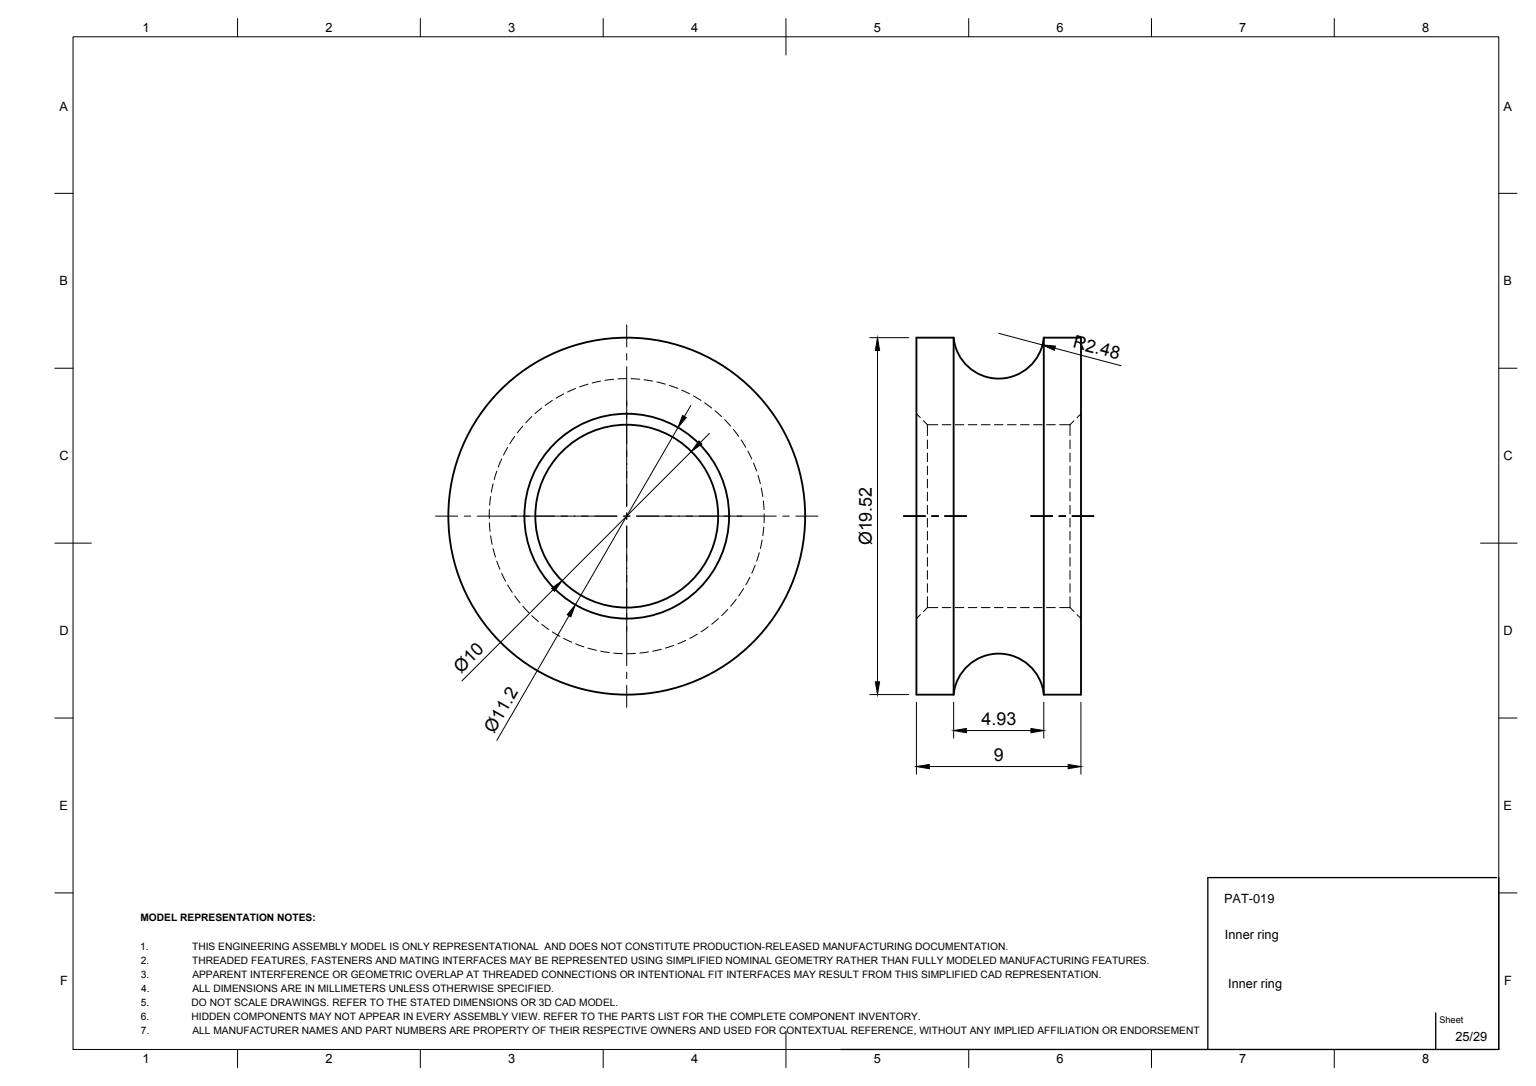
ISO-10303-21;
HEADER;
/* Generated by software containing ST-Developer
 * from STEP Tools, Inc. (www.steptools.com) 
 */

FILE_DESCRIPTION(
/* description */ ('Caster wheel assembly'),
/* implementation_level */ '2;1');

FILE_NAME(
/* name */ 'Inner ring.step',
/* time_stamp */ '2026-10-28T03:23:56-07:00',
/* author */ (''),
/* organization */ (''),
/* preprocessor_version */ 'ST-DEVELOPER v20.2',
/* originating_system */ 'Autodesk Translation Framework v15.17.0.0',
/* authorisation */ '');

FILE_SCHEMA (('AUTOMOTIVE_DESIGN { 1 0 10303 214 3 1 1 }'));
ENDSEC;

DATA;
#10=MECHANICAL_DESIGN_GEOMETRIC_PRESENTATION_REPRESENTATION('',(#239),#5385);
#45=TOROIDAL_SURFACE('',#3164,1.,0.247676);
#174=CONICAL_SURFACE('',#3175,0.53,0.785398163397448);
#175=CONICAL_SURFACE('',#3182,0.53,0.785398163397448);
#195=SHAPE_REPRESENTATION_RELATIONSHIP('SRR','None',#5493,#217);
#217=ADVANCED_BREP_SHAPE_REPRESENTATION('',(#268),#5380);
#239=STYLED_ITEM('',(#5672),#268);
#268=MANIFOLD_SOLID_BREP('Body1',#2667);
#324=FACE_BOUND('',#754,.T.);
#325=FACE_BOUND('',#757,.T.);
#404=PLANE('',#3177);
#405=PLANE('',#3180);
#538=FACE_OUTER_BOUND('',#749,.T.);
#539=FACE_OUTER_BOUND('',#750,.T.);
#540=FACE_OUTER_BOUND('',#751,.T.);
#541=FACE_OUTER_BOUND('',#752,.T.);
#542=FACE_OUTER_BOUND('',#753,.T.);
#543=FACE_OUTER_BOUND('',#755,.T.);
#544=FACE_OUTER_BOUND('',#756,.T.);
#545=FACE_OUTER_BOUND('',#758,.T.);
#749=EDGE_LOOP('',(#2216,#2217,#2218,#2219,#2220,#2221));
#750=EDGE_LOOP('',(#2222,#2223,#2224,#2225,#2226));
#751=EDGE_LOOP('',(#2227,#2228,#2229,#2230));
#752=EDGE_LOOP('',(#2231,#2232,#2233,#2234));
#753=EDGE_LOOP('',(#2235));
#754=EDGE_LOOP('',(#2236));
#755=EDGE_LOOP('',(#2237,#2238,#2239,#2240,#2241));
#756=EDGE_LOOP('',(#2242));
#757=EDGE_LOOP('',(#2243));
#758=EDGE_LOOP('',(#2244,#2245,#2246,#2247));
#927=LINE('',#4750,#1061);
#928=LINE('',#4756,#1062);
#929=LINE('',#4760,#1063);
#930=LINE('',#4766,#1064);
#931=LINE('',#4771,#1065);
#1061=VECTOR('',#3918,0.976185);
#1062=VECTOR('',#3925,0.5);
#1063=VECTOR('',#3930,0.53);
#1064=VECTOR('',#3939,0.976185);
#1065=VECTOR('',#3946,0.53);
#1164=CIRCLE('',#3165,0.976185);
#1165=CIRCLE('',#3166,0.976185);
#1166=CIRCLE('',#3167,0.247676);
#1167=CIRCLE('',#3168,0.976185);
#1168=CIRCLE('',#3169,0.976185);
#1169=CIRCLE('',#3171,0.976185);
#1170=CIRCLE('',#3173,0.5);
#1171=CIRCLE('',#3174,0.5);
#1172=CIRCLE('',#3176,0.56);
#1173=CIRCLE('',#3179,0.976185);
#1174=CIRCLE('',#3181,0.56);
#1379=VERTEX_POINT('',#4739);
#1380=VERTEX_POINT('',#4740);
#1381=VERTEX_POINT('',#4743);
#1382=VERTEX_POINT('',#4745);
#1383=VERTEX_POINT('',#4749);
#1384=VERTEX_POINT('',#4753);
#1385=VERTEX_POINT('',#4755);
#1386=VERTEX_POINT('',#4759);
#1387=VERTEX_POINT('',#4764);
#1388=VERTEX_POINT('',#4768);
#1676=EDGE_CURVE('',#1379,#1380,#1164,.T.);
#1677=EDGE_CURVE('',#1380,#1379,#1165,.T.);
#1678=EDGE_CURVE('',#1380,#1381,#1166,.T.);
#1679=EDGE_CURVE('',#1382,#1381,#1167,.T.);
#1680=EDGE_CURVE('',#1381,#1382,#1168,.T.);
#1681=EDGE_CURVE('',#1382,#1383,#927,.T.);
#1682=EDGE_CURVE('',#1383,#1383,#1169,.T.);
#1683=EDGE_CURVE('',#1384,#1384,#1170,.T.);
#1684=EDGE_CURVE('',#1384,#1385,#928,.T.);
#1685=EDGE_CURVE('',#1385,#1385,#1171,.T.);
#1686=EDGE_CURVE('',#1385,#1386,#929,.T.);
#1687=EDGE_CURVE('',#1386,#1386,#1172,.T.);
#1688=EDGE_CURVE('',#1387,#1387,#1173,.T.);
#1689=EDGE_CURVE('',#1387,#1379,#930,.T.);
#1690=EDGE_CURVE('',#1388,#1388,#1174,.T.);
#1691=EDGE_CURVE('',#1388,#1384,#931,.T.);
#2216=ORIENTED_EDGE('',*,*,#1676,.F.);
#2217=ORIENTED_EDGE('',*,*,#1677,.F.);
#2218=ORIENTED_EDGE('',*,*,#1678,.T.);
#2219=ORIENTED_EDGE('',*,*,#1679,.F.);
#2220=ORIENTED_EDGE('',*,*,#1680,.F.);
#2221=ORIENTED_EDGE('',*,*,#1678,.F.);
#2222=ORIENTED_EDGE('',*,*,#1679,.T.);
#2223=ORIENTED_EDGE('',*,*,#1680,.T.);
#2224=ORIENTED_EDGE('',*,*,#1681,.T.);
#2225=ORIENTED_EDGE('',*,*,#1682,.T.);
#2226=ORIENTED_EDGE('',*,*,#1681,.F.);
#2227=ORIENTED_EDGE('',*,*,#1683,.T.);
#2228=ORIENTED_EDGE('',*,*,#1684,.T.);
#2229=ORIENTED_EDGE('',*,*,#1685,.F.);
#2230=ORIENTED_EDGE('',*,*,#1684,.F.);
#2231=ORIENTED_EDGE('',*,*,#1685,.T.);
#2232=ORIENTED_EDGE('',*,*,#1686,.T.);
#2233=ORIENTED_EDGE('',*,*,#1687,.F.);
#2234=ORIENTED_EDGE('',*,*,#1686,.F.);
#2235=ORIENTED_EDGE('',*,*,#1682,.F.);
#2236=ORIENTED_EDGE('',*,*,#1687,.T.);
#2237=ORIENTED_EDGE('',*,*,#1688,.F.);
#2238=ORIENTED_EDGE('',*,*,#1689,.T.);
#2239=ORIENTED_EDGE('',*,*,#1676,.T.);
#2240=ORIENTED_EDGE('',*,*,#1677,.T.);
#2241=ORIENTED_EDGE('',*,*,#1689,.F.);
#2242=ORIENTED_EDGE('',*,*,#1688,.T.);
#2243=ORIENTED_EDGE('',*,*,#1690,.F.);
#2244=ORIENTED_EDGE('',*,*,#1690,.T.);
#2245=ORIENTED_EDGE('',*,*,#1691,.T.);
#2246=ORIENTED_EDGE('',*,*,#1683,.F.);
#2247=ORIENTED_EDGE('',*,*,#1691,.F.);
#2469=CYLINDRICAL_SURFACE('',#3170,0.976185);
#2470=CYLINDRICAL_SURFACE('',#3172,0.5);
#2471=CYLINDRICAL_SURFACE('',#3178,0.976185);
#2598=ADVANCED_FACE('',(#538),#45,.F.);
#2599=ADVANCED_FACE('',(#539),#2469,.T.);
#2600=ADVANCED_FACE('',(#540),#2470,.F.);
#2601=ADVANCED_FACE('',(#541),#174,.F.);
#2602=ADVANCED_FACE('',(#542,#324),#404,.T.);
#2603=ADVANCED_FACE('',(#543),#2471,.T.);
#2604=ADVANCED_FACE('',(#544,#325),#405,.T.);
#2605=ADVANCED_FACE('',(#545),#175,.F.);
#2667=CLOSED_SHELL('',(#2598,#2599,#2600,#2601,#2602,#2603,#2604,#2605));
#3163=AXIS2_PLACEMENT_3D('',#4737,#3902,#3903);
#3164=AXIS2_PLACEMENT_3D('',#4738,#3904,#3905);
#3165=AXIS2_PLACEMENT_3D('',#4741,#3906,#3907);
#3166=AXIS2_PLACEMENT_3D('',#4742,#3908,#3909);
#3167=AXIS2_PLACEMENT_3D('',#4744,#3910,#3911);
#3168=AXIS2_PLACEMENT_3D('',#4746,#3912,#3913);
#3169=AXIS2_PLACEMENT_3D('',#4747,#3914,#3915);
#3170=AXIS2_PLACEMENT_3D('',#4748,#3916,#3917);
#3171=AXIS2_PLACEMENT_3D('',#4751,#3919,#3920);
#3172=AXIS2_PLACEMENT_3D('',#4752,#3921,#3922);
#3173=AXIS2_PLACEMENT_3D('',#4754,#3923,#3924);
#3174=AXIS2_PLACEMENT_3D('',#4757,#3926,#3927);
#3175=AXIS2_PLACEMENT_3D('',#4758,#3928,#3929);
#3176=AXIS2_PLACEMENT_3D('',#4761,#3931,#3932);
#3177=AXIS2_PLACEMENT_3D('',#4762,#3933,#3934);
#3178=AXIS2_PLACEMENT_3D('',#4763,#3935,#3936);
#3179=AXIS2_PLACEMENT_3D('',#4765,#3937,#3938);
#3180=AXIS2_PLACEMENT_3D('',#4767,#3940,#3941);
#3181=AXIS2_PLACEMENT_3D('',#4769,#3942,#3943);
#3182=AXIS2_PLACEMENT_3D('',#4770,#3944,#3945);
#3902=DIRECTION('axis',(0.,0.,1.));
#3903=DIRECTION('refdir',(1.,0.,0.));
#3904=DIRECTION('center_axis',(0.,-1.,0.));
#3905=DIRECTION('ref_axis',(0.,0.,-1.));
#3906=DIRECTION('center_axis',(0.,-1.,0.));
#3907=DIRECTION('ref_axis',(1.,0.,0.));
#3908=DIRECTION('center_axis',(0.,-1.,0.));
#3909=DIRECTION('ref_axis',(1.,0.,0.));
#3910=DIRECTION('center_axis',(1.,0.,1.22464679914735E-16));
#3911=DIRECTION('ref_axis',(-1.22464679914735E-16,0.,1.));
#3912=DIRECTION('center_axis',(0.,1.,0.));
#3913=DIRECTION('ref_axis',(1.,0.,0.));
#3914=DIRECTION('center_axis',(0.,1.,0.));
#3915=DIRECTION('ref_axis',(1.,0.,0.));
#3916=DIRECTION('center_axis',(0.,-1.,0.));
#3917=DIRECTION('ref_axis',(1.,0.,0.));
#3918=DIRECTION('',(0.,1.,0.));
#3919=DIRECTION('center_axis',(0.,-1.,0.));
#3920=DIRECTION('ref_axis',(1.,0.,0.));
#3921=DIRECTION('center_axis',(0.,-1.,0.));
#3922=DIRECTION('ref_axis',(1.,0.,0.));
#3923=DIRECTION('center_axis',(0.,-1.,0.));
#3924=DIRECTION('ref_axis',(1.,0.,0.));
#3925=DIRECTION('',(0.,1.,0.));
#3926=DIRECTION('center_axis',(0.,-1.,0.));
#3927=DIRECTION('ref_axis',(1.,0.,0.));
#3928=DIRECTION('center_axis',(0.,1.,0.));
#3929=DIRECTION('ref_axis',(1.,0.,0.));
#3930=DIRECTION('',(-0.707106781186547,0.707106781186548,-8.65956056235493E-17));
#3931=DIRECTION('center_axis',(0.,-1.,0.));
#3932=DIRECTION('ref_axis',(1.,0.,0.));
#3933=DIRECTION('center_axis',(0.,1.,0.));
#3934=DIRECTION('ref_axis',(0.,0.,1.));
#3935=DIRECTION('center_axis',(0.,-1.,0.));
#3936=DIRECTION('ref_axis',(1.,0.,0.));
#3937=DIRECTION('center_axis',(0.,-1.,0.));
#3938=DIRECTION('ref_axis',(1.,0.,0.));
#3939=DIRECTION('',(0.,1.,0.));
#3940=DIRECTION('center_axis',(0.,-1.,0.));
#3941=DIRECTION('ref_axis',(0.,0.,-1.));
#3942=DIRECTION('center_axis',(0.,-1.,0.));
#3943=DIRECTION('ref_axis',(1.,0.,0.));
#3944=DIRECTION('center_axis',(0.,-1.,0.));
#3945=DIRECTION('ref_axis',(1.,0.,0.));
#3946=DIRECTION('',(0.707106781186547,0.707106781186548,8.65956056235493E-17));
#4737=CARTESIAN_POINT('',(0.,0.,0.));
#4738=CARTESIAN_POINT('Origin',(0.,0.,0.));
#4739=CARTESIAN_POINT('',(-0.976185,-0.246528389340863,-1.19548183562566E-16));
#4740=CARTESIAN_POINT('',(-1.19548183562566E-16,-0.246528389340863,0.976185));
#4741=CARTESIAN_POINT('Origin',(0.,-0.246528389340863,0.));
#4742=CARTESIAN_POINT('Origin',(0.,-0.246528389340863,0.));
#4743=CARTESIAN_POINT('',(-1.19548183562566E-16,0.246528389340863,0.976185));
#4744=CARTESIAN_POINT('Origin',(-1.22464679914735E-16,0.,1.));
#4745=CARTESIAN_POINT('',(-0.976185,0.246528389340863,1.19548183562566E-16));
#4746=CARTESIAN_POINT('Origin',(0.,0.246528389340863,0.));
#4747=CARTESIAN_POINT('Origin',(0.,0.246528389340863,0.));
#4748=CARTESIAN_POINT('Origin',(0.,0.,0.));
#4749=CARTESIAN_POINT('',(-0.976185,0.45,-1.19548183562566E-16));
#4750=CARTESIAN_POINT('',(-0.976185,0.,-1.19548183562566E-16));
#4751=CARTESIAN_POINT('Origin',(0.,0.45,0.));
#4752=CARTESIAN_POINT('Origin',(0.,0.,0.));
#4753=CARTESIAN_POINT('',(-0.5,-0.39,-6.12323399573677E-17));
#4754=CARTESIAN_POINT('Origin',(0.,-0.39,0.));
#4755=CARTESIAN_POINT('',(-0.5,0.39,-6.12323399573677E-17));
#4756=CARTESIAN_POINT('',(-0.5,0.,-6.12323399573677E-17));
#4757=CARTESIAN_POINT('Origin',(0.,0.39,0.));
#4758=CARTESIAN_POINT('Origin',(0.,0.42,0.));
#4759=CARTESIAN_POINT('',(-0.56,0.45,-6.85802207522518E-17));
#4760=CARTESIAN_POINT('',(-0.53,0.42,-6.49062803548097E-17));
#4761=CARTESIAN_POINT('Origin',(0.,0.45,0.));
#4762=CARTESIAN_POINT('Origin',(0.976185,0.45,0.));
#4763=CARTESIAN_POINT('Origin',(0.,0.,0.));
#4764=CARTESIAN_POINT('',(-0.976185,-0.45,-1.19548183562566E-16));
#4765=CARTESIAN_POINT('Origin',(0.,-0.45,0.));
#4766=CARTESIAN_POINT('',(-0.976185,0.,-1.19548183562566E-16));
#4767=CARTESIAN_POINT('Origin',(0.56,-0.45,0.));
#4768=CARTESIAN_POINT('',(-0.56,-0.45,-6.85802207522518E-17));
#4769=CARTESIAN_POINT('Origin',(0.,-0.45,0.));
#4770=CARTESIAN_POINT('Origin',(0.,-0.42,0.));
#4771=CARTESIAN_POINT('',(-0.53,-0.42,-6.49062803548097E-17));
#5352=UNCERTAINTY_MEASURE_WITH_UNIT(LENGTH_MEASURE(0.001),#5386,
'DISTANCE_ACCURACY_VALUE',
'Maximum model space distance between geometric entities at asserted c
onnectivities');
#5357=UNCERTAINTY_MEASURE_WITH_UNIT(LENGTH_MEASURE(0.001),#5386,
'DISTANCE_ACCURACY_VALUE',
'Maximum model space distance between geometric entities at asserted c
onnectivities');
#5380=(
GEOMETRIC_REPRESENTATION_CONTEXT(3)
GLOBAL_UNCERTAINTY_ASSIGNED_CONTEXT((#5352))
GLOBAL_UNIT_ASSIGNED_CONTEXT((#5386,#5388,#5389))
REPRESENTATION_CONTEXT('','3D')
);
#5385=(
GEOMETRIC_REPRESENTATION_CONTEXT(3)
GLOBAL_UNCERTAINTY_ASSIGNED_CONTEXT((#5357))
GLOBAL_UNIT_ASSIGNED_CONTEXT((#5386,#5388,#5389))
REPRESENTATION_CONTEXT('','3D')
);
#5386=(
LENGTH_UNIT()
NAMED_UNIT(*)
SI_UNIT(.CENTI.,.METRE.)
);
#5388=(
NAMED_UNIT(*)
PLANE_ANGLE_UNIT()
SI_UNIT($,.RADIAN.)
);
#5389=(
NAMED_UNIT(*)
SI_UNIT($,.STERADIAN.)
SOLID_ANGLE_UNIT()
);
#5412=SHAPE_DEFINITION_REPRESENTATION(#5453,#5493);
#5453=PRODUCT_DEFINITION_SHAPE('',$,#5521);
#5493=SHAPE_REPRESENTATION('',(#3163),#5380);
#5498=PRODUCT_DEFINITION_CONTEXT('part definition',#5581,'design');
#5521=PRODUCT_DEFINITION('Inner ring','Inner ring',#5548,#5498);
#5548=PRODUCT_DEFINITION_FORMATION('',$,#5605);
#5581=APPLICATION_CONTEXT(
'Core Data for Automotive Mechanical Design Process');
#5582=PRODUCT_CONTEXT('part definition',#5581,'mechanical');
#5605=PRODUCT('Inner ring','Inner ring','Inner ring',(#5582));
#5666=COLOUR_RGB('Grey',0.48,0.52,0.57);
#5667=FILL_AREA_STYLE_COLOUR('',#5666);
#5668=FILL_AREA_STYLE('',(#5667));
#5669=SURFACE_STYLE_FILL_AREA(#5668);
#5670=SURFACE_SIDE_STYLE('',(#5669));
#5671=SURFACE_STYLE_USAGE(.BOTH.,#5670);
#5672=PRESENTATION_STYLE_ASSIGNMENT((#5671));
ENDSEC;
END-ISO-10303-21;
